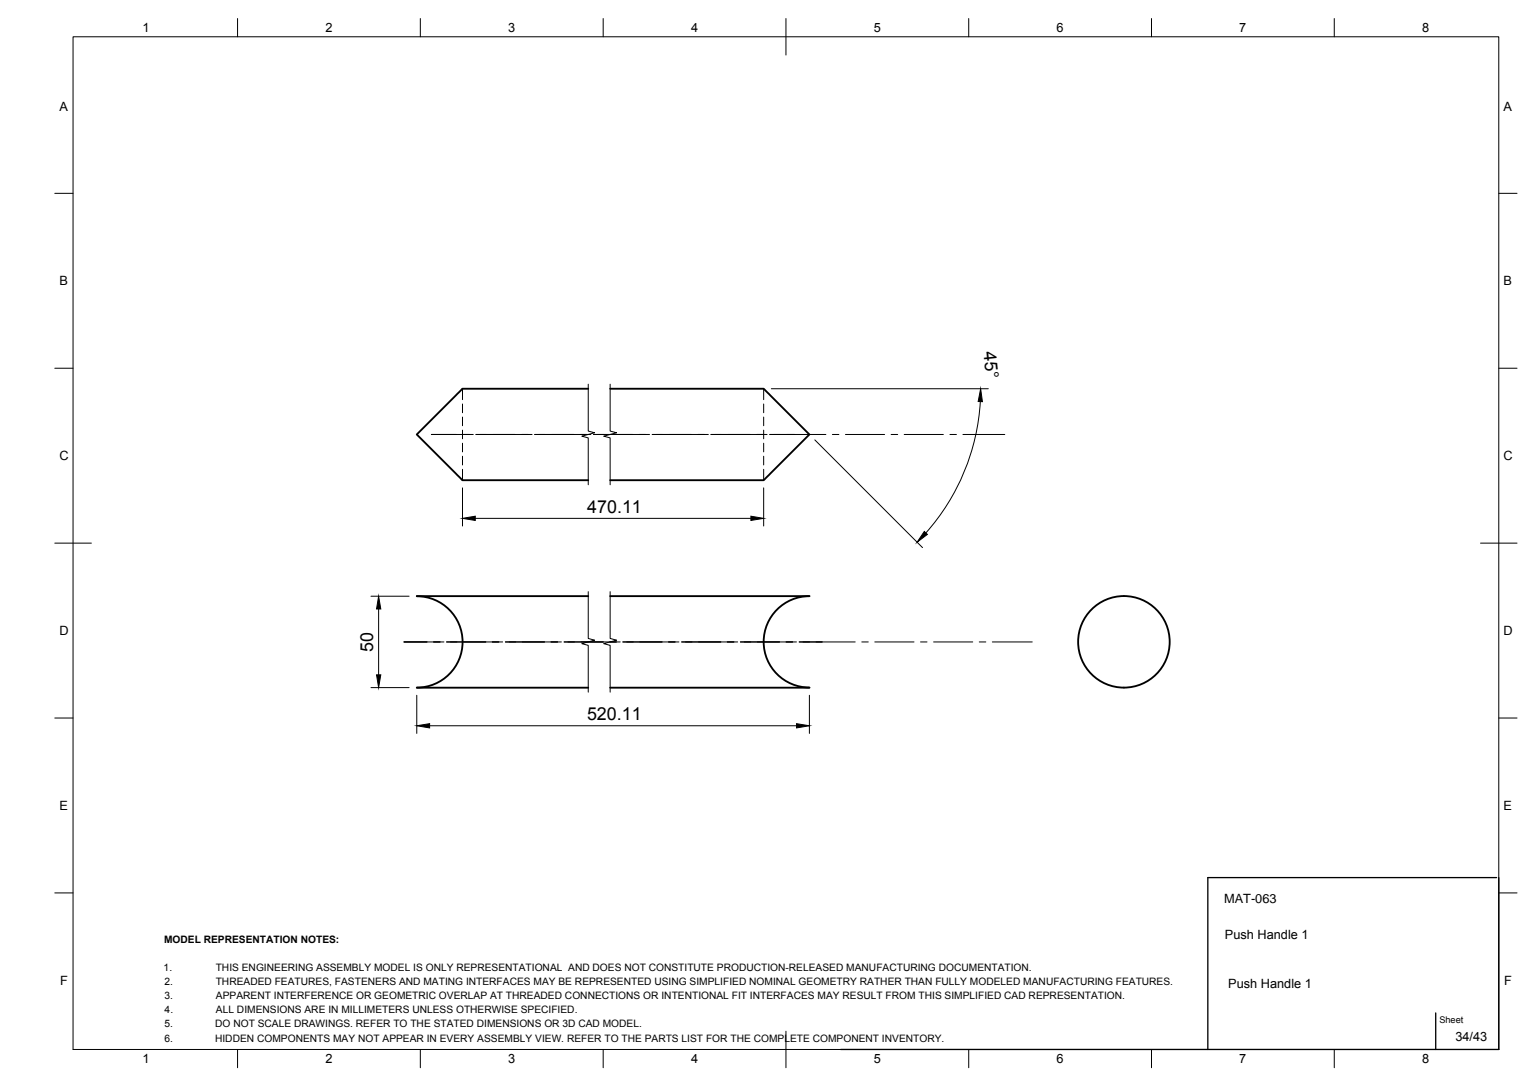
ISO-10303-21;
HEADER;
/* Generated by software containing ST-Developer
 * from STEP Tools, Inc. (www.steptools.com) 
 */

FILE_DESCRIPTION(
/* description */ (''),
/* implementation_level */ '2;1');

FILE_NAME(
/* name */ 'Push Handle 1.step',
/* time_stamp */ '2026-10-24T09:43:01-07:00',
/* author */ (''),
/* organization */ (''),
/* preprocessor_version */ 'ST-DEVELOPER v20.2',
/* originating_system */ 'Autodesk Translation Framework v15.15.0.0',
/* authorisation */ '');

FILE_SCHEMA (('AUTOMOTIVE_DESIGN { 1 0 10303 214 3 1 1 }'));
ENDSEC;

DATA;
#10=MECHANICAL_DESIGN_GEOMETRIC_PRESENTATION_REPRESENTATION('',(#297),#11112);
#11=ELLIPSE('',#7146,0.035355338987388,0.0249999999491312);
#12=ELLIPSE('',#7147,0.0353553389873879,0.0249999999491312);
#13=ELLIPSE('',#7149,0.0353553389873867,0.0249999999491303);
#14=ELLIPSE('',#7150,0.0353553389873867,0.0249999999491303);
#231=SHAPE_REPRESENTATION_RELATIONSHIP('SRR','None',#11257,#264);
#264=ADVANCED_BREP_SHAPE_REPRESENTATION('',(#330),#11102);
#297=STYLED_ITEM('',(#11426),#330);
#330=MANIFOLD_SOLID_BREP('Push Handle 1',#6034);
#997=FACE_OUTER_BOUND('',#1501,.T.);
#998=FACE_OUTER_BOUND('',#1502,.T.);
#999=FACE_OUTER_BOUND('',#1503,.T.);
#1501=EDGE_LOOP('',(#5365,#5366));
#1502=EDGE_LOOP('',(#5367,#5368,#5369,#5370,#5371,#5372));
#1503=EDGE_LOOP('',(#5373,#5374));
#1892=LINE('',#10856,#2251);
#2251=VECTOR('',#9078,0.0249999998982604);
#3134=VERTEX_POINT('',#10850);
#3135=VERTEX_POINT('',#10851);
#3136=VERTEX_POINT('',#10855);
#3137=VERTEX_POINT('',#10857);
#3886=EDGE_CURVE('',#3134,#3135,#11,.T.);
#3887=EDGE_CURVE('',#3135,#3134,#12,.F.);
#3888=EDGE_CURVE('',#3135,#3136,#1892,.T.);
#3889=EDGE_CURVE('',#3136,#3137,#13,.F.);
#3890=EDGE_CURVE('',#3137,#3136,#14,.T.);
#5365=ORIENTED_EDGE('',*,*,#3886,.F.);
#5366=ORIENTED_EDGE('',*,*,#3887,.F.);
#5367=ORIENTED_EDGE('',*,*,#3887,.T.);
#5368=ORIENTED_EDGE('',*,*,#3886,.T.);
#5369=ORIENTED_EDGE('',*,*,#3888,.T.);
#5370=ORIENTED_EDGE('',*,*,#3889,.T.);
#5371=ORIENTED_EDGE('',*,*,#3890,.T.);
#5372=ORIENTED_EDGE('',*,*,#3888,.F.);
#5373=ORIENTED_EDGE('',*,*,#3890,.F.);
#5374=ORIENTED_EDGE('',*,*,#3889,.F.);
#5623=CYLINDRICAL_SURFACE('',#7145,0.0250000000000019);
#5624=CYLINDRICAL_SURFACE('',#7148,0.0249999998982604);
#5625=CYLINDRICAL_SURFACE('',#7151,0.025);
#5970=ADVANCED_FACE('',(#997),#5623,.F.);
#5971=ADVANCED_FACE('',(#998),#5624,.T.);
#5972=ADVANCED_FACE('',(#999),#5625,.F.);
#6034=CLOSED_SHELL('',(#5970,#5971,#5972));
#7144=AXIS2_PLACEMENT_3D('',#10848,#9068,#9069);
#7145=AXIS2_PLACEMENT_3D('',#10849,#9070,#9071);
#7146=AXIS2_PLACEMENT_3D('',#10852,#9072,#9073);
#7147=AXIS2_PLACEMENT_3D('',#10853,#9074,#9075);
#7148=AXIS2_PLACEMENT_3D('',#10854,#9076,#9077);
#7149=AXIS2_PLACEMENT_3D('',#10858,#9079,#9080);
#7150=AXIS2_PLACEMENT_3D('',#10859,#9081,#9082);
#7151=AXIS2_PLACEMENT_3D('',#10860,#9083,#9084);
#9068=DIRECTION('axis',(0.,0.,1.));
#9069=DIRECTION('refdir',(1.,0.,0.));
#9070=DIRECTION('center_axis',(1.,0.,2.22044604925031E-15));
#9071=DIRECTION('ref_axis',(2.22044604925031E-15,0.,-1.));
#9072=DIRECTION('center_axis',(0.707106781186548,0.530215432236494,-0.467837146257399));
#9073=DIRECTION('ref_axis',(0.707106781186547,-0.530215432236493,0.467837146257402));
#9074=DIRECTION('center_axis',(0.707106781186547,-0.530215432236493,0.467837146257402));
#9075=DIRECTION('ref_axis',(0.707106781186548,0.530215432236494,-0.467837146257399));
#9076=DIRECTION('center_axis',(0.,-0.749837855248362,0.661621637219141));
#9077=DIRECTION('ref_axis',(0.,-0.661621637219141,-0.749837855248362));
#9078=DIRECTION('',(0.,0.749837855248362,-0.661621637219141));
#9079=DIRECTION('center_axis',(-0.707106781186548,0.530215432236494,-0.4678371462574));
#9080=DIRECTION('ref_axis',(-0.707106781186547,-0.530215432236494,0.4678371462574));
#9081=DIRECTION('center_axis',(-0.707106781186548,-0.530215432236494,0.4678371462574));
#9082=DIRECTION('ref_axis',(-0.707106781186547,0.530215432236494,-0.4678371462574));
#9083=DIRECTION('center_axis',(-1.,0.,0.));
#9084=DIRECTION('ref_axis',(0.,0.,1.));
#10848=CARTESIAN_POINT('',(0.,0.,0.));
#10849=CARTESIAN_POINT('Origin',(-0.560710678,0.3,-0.955882353));
#10850=CARTESIAN_POINT('',(0.3,0.283459459165354,-0.974628299273763));
#10851=CARTESIAN_POINT('',(0.29999999999996,0.316540540959,-0.937136406587632));
#10852=CARTESIAN_POINT('Origin',(0.3,0.300000000061598,-0.955882352930187));
#10853=CARTESIAN_POINT('Origin',(0.3,0.300000000061598,-0.955882352930187));
#10854=CARTESIAN_POINT('Origin',(0.3,0.716460202,-1.323347237));
#10855=CARTESIAN_POINT('',(0.29999999999999,0.706540540912883,-1.28125405363754));
#10856=CARTESIAN_POINT('',(0.3,0.733000742863165,-1.30460129069508));
#10857=CARTESIAN_POINT('',(0.299999999999999,0.673459459119104,-1.31874594632356));
#10858=CARTESIAN_POINT('Origin',(0.3,0.690000000016651,-1.29999999998113));
#10859=CARTESIAN_POINT('Origin',(0.3,0.690000000016651,-1.29999999998113));
#10860=CARTESIAN_POINT('Origin',(0.35,0.69,-1.3));
#11063=UNCERTAINTY_MEASURE_WITH_UNIT(LENGTH_MEASURE(1.E-5),#11113,
'DISTANCE_ACCURACY_VALUE',
'Maximum model space distance between geometric entities at asserted c
onnectivities');
#11073=UNCERTAINTY_MEASURE_WITH_UNIT(LENGTH_MEASURE(1.E-5),#11113,
'DISTANCE_ACCURACY_VALUE',
'Maximum model space distance between geometric entities at asserted c
onnectivities');
#11102=(
GEOMETRIC_REPRESENTATION_CONTEXT(3)
GLOBAL_UNCERTAINTY_ASSIGNED_CONTEXT((#11063))
GLOBAL_UNIT_ASSIGNED_CONTEXT((#11113,#11114,#11115))
REPRESENTATION_CONTEXT('','3D')
);
#11112=(
GEOMETRIC_REPRESENTATION_CONTEXT(3)
GLOBAL_UNCERTAINTY_ASSIGNED_CONTEXT((#11073))
GLOBAL_UNIT_ASSIGNED_CONTEXT((#11113,#11114,#11115))
REPRESENTATION_CONTEXT('','3D')
);
#11113=(
LENGTH_UNIT()
NAMED_UNIT(*)
SI_UNIT($,.METRE.)
);
#11114=(
NAMED_UNIT(*)
PLANE_ANGLE_UNIT()
SI_UNIT($,.RADIAN.)
);
#11115=(
NAMED_UNIT(*)
SI_UNIT($,.STERADIAN.)
SOLID_ANGLE_UNIT()
);
#11144=SHAPE_DEFINITION_REPRESENTATION(#11195,#11257);
#11195=PRODUCT_DEFINITION_SHAPE('',$,#11296);
#11257=SHAPE_REPRESENTATION('',(#7144),#11102);
#11267=PRODUCT_DEFINITION_CONTEXT('part definition',#11383,'design');
#11296=PRODUCT_DEFINITION('Push Handle 1','Push Handle 1',#11334,#11267);
#11334=PRODUCT_DEFINITION_FORMATION('',$,#11413);
#11383=APPLICATION_CONTEXT(
'Core Data for Automotive Mechanical Design Process');
#11384=PRODUCT_CONTEXT('part definition',#11383,'mechanical');
#11413=PRODUCT('Push Handle 1','Push Handle 1',
'back_push__ DE     2693',(#11384));
#11426=PRESENTATION_STYLE_ASSIGNMENT((#11430));
#11430=SURFACE_STYLE_USAGE(.BOTH.,#11434);
#11434=SURFACE_SIDE_STYLE('',(#11438));
#11438=SURFACE_STYLE_FILL_AREA(#11442);
#11442=FILL_AREA_STYLE('Opaque(202,209,238)',(#11446));
#11446=FILL_AREA_STYLE_COLOUR('Opaque(202,209,238)',#11450);
#11450=COLOUR_RGB('Opaque(202,209,238)',0.792156862745098,0.819607843137255,
0.933333333333333);
ENDSEC;
END-ISO-10303-21;
